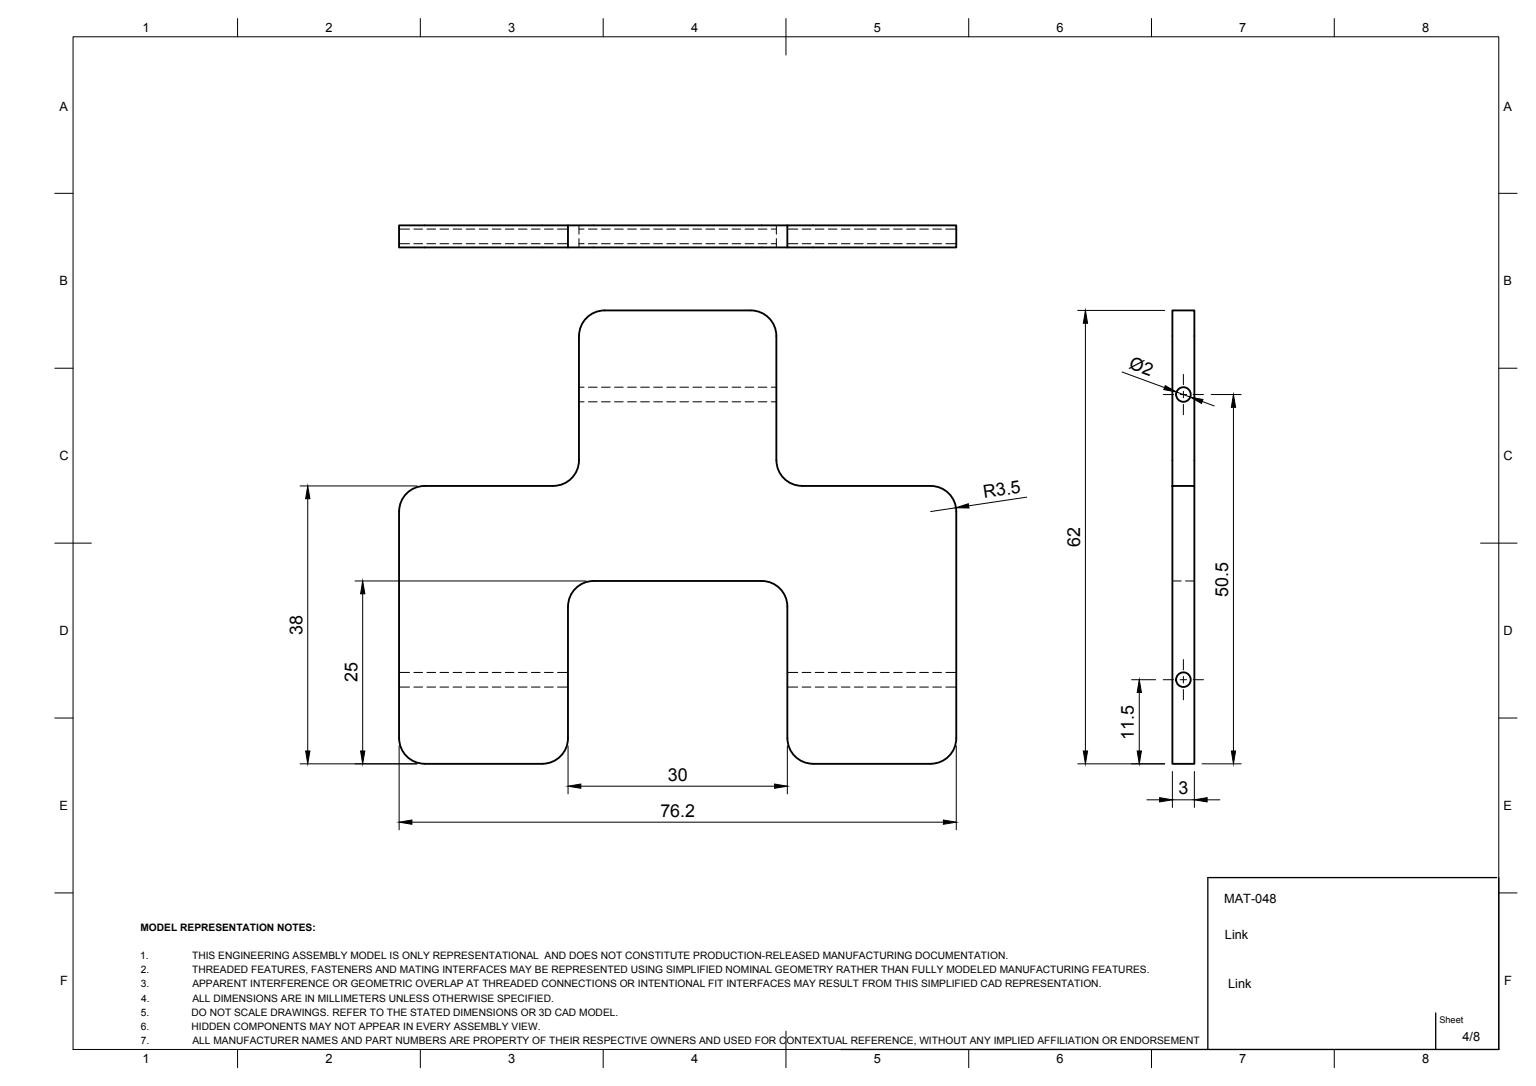
ISO-10303-21;
HEADER;
/* Generated by software containing ST-Developer
 * from STEP Tools, Inc. (www.steptools.com) 
 */

FILE_DESCRIPTION(
/* description */ ('STEP AP214'),
/* implementation_level */ '2;1');

FILE_NAME(
/* name */ 'Link.step',
/* time_stamp */ '2026-11-14T22:24:45-08:00',
/* author */ (''),
/* organization */ (''),
/* preprocessor_version */ 'ST-DEVELOPER v20.2',
/* originating_system */ 'Autodesk Translation Framework v15.17.0.0',
/* authorisation */ '');

FILE_SCHEMA (('AUTOMOTIVE_DESIGN { 1 0 10303 214 3 1 1 }'));
ENDSEC;

DATA;
#10=MECHANICAL_DESIGN_GEOMETRIC_PRESENTATION_REPRESENTATION('',(#129),#5599);
#107=FACE_BOUND('',#614,.T.);
#108=FACE_BOUND('',#619,.T.);
#109=FACE_BOUND('',#624,.T.);
#110=FACE_BOUND('',#629,.T.);
#111=FACE_BOUND('',#634,.T.);
#112=FACE_BOUND('',#639,.T.);
#117=SHAPE_REPRESENTATION_RELATIONSHIP('SRR','None',#5645,#123);
#123=ADVANCED_BREP_SHAPE_REPRESENTATION('',(#135),#5597);
#129=STYLED_ITEM('',(#5680),#135);
#135=MANIFOLD_SOLID_BREP('Body1',#3311);
#177=CYLINDRICAL_SURFACE('',#3594,0.999999999999991);
#178=CYLINDRICAL_SURFACE('',#3597,0.999999999999991);
#179=CYLINDRICAL_SURFACE('',#3600,1.);
#180=CYLINDRICAL_SURFACE('',#3603,3.5);
#181=CYLINDRICAL_SURFACE('',#3607,3.5);
#182=CYLINDRICAL_SURFACE('',#3611,3.5);
#183=CYLINDRICAL_SURFACE('',#3615,3.5);
#184=CYLINDRICAL_SURFACE('',#3619,3.5);
#185=CYLINDRICAL_SURFACE('',#3623,3.5);
#186=CYLINDRICAL_SURFACE('',#3627,3.5);
#187=CYLINDRICAL_SURFACE('',#3631,3.5);
#188=CYLINDRICAL_SURFACE('',#3635,3.5);
#189=CYLINDRICAL_SURFACE('',#3639,3.5);
#190=CYLINDRICAL_SURFACE('',#3643,3.5);
#191=CYLINDRICAL_SURFACE('',#3647,3.5);
#249=CIRCLE('',#3595,0.999999999999991);
#250=CIRCLE('',#3596,0.999999999999991);
#251=CIRCLE('',#3598,0.999999999999991);
#252=CIRCLE('',#3599,0.999999999999991);
#253=CIRCLE('',#3601,0.999999999999988);
#254=CIRCLE('',#3602,1.);
#255=CIRCLE('',#3604,3.5);
#256=CIRCLE('',#3605,3.5);
#257=CIRCLE('',#3608,3.5);
#258=CIRCLE('',#3609,3.5);
#259=CIRCLE('',#3612,3.5);
#260=CIRCLE('',#3613,3.5);
#261=CIRCLE('',#3616,3.5);
#262=CIRCLE('',#3617,3.5);
#263=CIRCLE('',#3620,3.5);
#264=CIRCLE('',#3621,3.5);
#265=CIRCLE('',#3624,3.5);
#266=CIRCLE('',#3625,3.5);
#267=CIRCLE('',#3628,3.5);
#268=CIRCLE('',#3629,3.5);
#269=CIRCLE('',#3632,3.5);
#270=CIRCLE('',#3633,3.5);
#271=CIRCLE('',#3636,3.5);
#272=CIRCLE('',#3637,3.5);
#273=CIRCLE('',#3640,3.5);
#274=CIRCLE('',#3641,3.5);
#275=CIRCLE('',#3644,3.5);
#276=CIRCLE('',#3645,3.5);
#277=CIRCLE('',#3648,3.5);
#278=CIRCLE('',#3649,3.5);
#425=FACE_OUTER_BOUND('',#609,.T.);
#426=FACE_OUTER_BOUND('',#610,.T.);
#427=FACE_OUTER_BOUND('',#611,.T.);
#428=FACE_OUTER_BOUND('',#612,.T.);
#429=FACE_OUTER_BOUND('',#613,.T.);
#430=FACE_OUTER_BOUND('',#615,.T.);
#431=FACE_OUTER_BOUND('',#616,.T.);
#432=FACE_OUTER_BOUND('',#617,.T.);
#433=FACE_OUTER_BOUND('',#618,.T.);
#434=FACE_OUTER_BOUND('',#620,.T.);
#435=FACE_OUTER_BOUND('',#621,.T.);
#436=FACE_OUTER_BOUND('',#622,.T.);
#437=FACE_OUTER_BOUND('',#623,.T.);
#438=FACE_OUTER_BOUND('',#625,.T.);
#439=FACE_OUTER_BOUND('',#626,.T.);
#440=FACE_OUTER_BOUND('',#627,.T.);
#441=FACE_OUTER_BOUND('',#628,.T.);
#442=FACE_OUTER_BOUND('',#630,.T.);
#443=FACE_OUTER_BOUND('',#631,.T.);
#444=FACE_OUTER_BOUND('',#632,.T.);
#445=FACE_OUTER_BOUND('',#633,.T.);
#446=FACE_OUTER_BOUND('',#635,.T.);
#447=FACE_OUTER_BOUND('',#636,.T.);
#448=FACE_OUTER_BOUND('',#637,.T.);
#449=FACE_OUTER_BOUND('',#638,.T.);
#450=FACE_OUTER_BOUND('',#640,.T.);
#451=FACE_OUTER_BOUND('',#641,.T.);
#452=FACE_OUTER_BOUND('',#642,.T.);
#453=FACE_OUTER_BOUND('',#643,.T.);
#609=EDGE_LOOP('',(#2835,#2836,#2837,#2838));
#610=EDGE_LOOP('',(#2839,#2840,#2841,#2842));
#611=EDGE_LOOP('',(#2843,#2844,#2845,#2846));
#612=EDGE_LOOP('',(#2847,#2848,#2849,#2850));
#613=EDGE_LOOP('',(#2851,#2852,#2853,#2854));
#614=EDGE_LOOP('',(#2855));
#615=EDGE_LOOP('',(#2856,#2857,#2858,#2859));
#616=EDGE_LOOP('',(#2860,#2861,#2862,#2863));
#617=EDGE_LOOP('',(#2864,#2865,#2866,#2867));
#618=EDGE_LOOP('',(#2868,#2869,#2870,#2871));
#619=EDGE_LOOP('',(#2872));
#620=EDGE_LOOP('',(#2873,#2874,#2875,#2876));
#621=EDGE_LOOP('',(#2877,#2878,#2879,#2880));
#622=EDGE_LOOP('',(#2881,#2882,#2883,#2884));
#623=EDGE_LOOP('',(#2885,#2886,#2887,#2888));
#624=EDGE_LOOP('',(#2889));
#625=EDGE_LOOP('',(#2890,#2891,#2892,#2893));
#626=EDGE_LOOP('',(#2894,#2895,#2896,#2897));
#627=EDGE_LOOP('',(#2898,#2899,#2900,#2901));
#628=EDGE_LOOP('',(#2902,#2903,#2904,#2905));
#629=EDGE_LOOP('',(#2906));
#630=EDGE_LOOP('',(#2907,#2908,#2909,#2910));
#631=EDGE_LOOP('',(#2911,#2912,#2913,#2914));
#632=EDGE_LOOP('',(#2915,#2916,#2917,#2918));
#633=EDGE_LOOP('',(#2919,#2920,#2921,#2922));
#634=EDGE_LOOP('',(#2923));
#635=EDGE_LOOP('',(#2924,#2925,#2926,#2927));
#636=EDGE_LOOP('',(#2928,#2929,#2930,#2931));
#637=EDGE_LOOP('',(#2932,#2933,#2934,#2935));
#638=EDGE_LOOP('',(#2936,#2937,#2938,#2939));
#639=EDGE_LOOP('',(#2940));
#640=EDGE_LOOP('',(#2941,#2942,#2943,#2944));
#641=EDGE_LOOP('',(#2945,#2946,#2947,#2948));
#642=EDGE_LOOP('',(#2949,#2950,#2951,#2952,#2953,#2954,#2955,#2956,#2957,
#2958,#2959,#2960,#2961,#2962,#2963,#2964,#2965,#2966,#2967,#2968,#2969,
#2970,#2971,#2972));
#643=EDGE_LOOP('',(#2973,#2974,#2975,#2976,#2977,#2978,#2979,#2980,#2981,
#2982,#2983,#2984,#2985,#2986,#2987,#2988,#2989,#2990,#2991,#2992,#2993,
#2994,#2995,#2996));
#951=LINE('',#5393,#1307);
#952=LINE('',#5399,#1308);
#953=LINE('',#5405,#1309);
#954=LINE('',#5412,#1310);
#955=LINE('',#5415,#1311);
#956=LINE('',#5418,#1312);
#957=LINE('',#5420,#1313);
#958=LINE('',#5421,#1314);
#959=LINE('',#5426,#1315);
#960=LINE('',#5430,#1316);
#961=LINE('',#5432,#1317);
#962=LINE('',#5433,#1318);
#963=LINE('',#5438,#1319);
#964=LINE('',#5442,#1320);
#965=LINE('',#5444,#1321);
#966=LINE('',#5445,#1322);
#967=LINE('',#5450,#1323);
#968=LINE('',#5454,#1324);
#969=LINE('',#5456,#1325);
#970=LINE('',#5457,#1326);
#971=LINE('',#5462,#1327);
#972=LINE('',#5466,#1328);
#973=LINE('',#5468,#1329);
#974=LINE('',#5469,#1330);
#975=LINE('',#5474,#1331);
#976=LINE('',#5478,#1332);
#977=LINE('',#5480,#1333);
#978=LINE('',#5481,#1334);
#979=LINE('',#5486,#1335);
#980=LINE('',#5490,#1336);
#981=LINE('',#5492,#1337);
#982=LINE('',#5493,#1338);
#983=LINE('',#5498,#1339);
#984=LINE('',#5502,#1340);
#985=LINE('',#5504,#1341);
#986=LINE('',#5505,#1342);
#987=LINE('',#5510,#1343);
#988=LINE('',#5514,#1344);
#989=LINE('',#5516,#1345);
#990=LINE('',#5517,#1346);
#991=LINE('',#5522,#1347);
#992=LINE('',#5526,#1348);
#993=LINE('',#5528,#1349);
#994=LINE('',#5529,#1350);
#995=LINE('',#5534,#1351);
#996=LINE('',#5538,#1352);
#997=LINE('',#5540,#1353);
#998=LINE('',#5541,#1354);
#999=LINE('',#5546,#1355);
#1000=LINE('',#5549,#1356);
#1001=LINE('',#5550,#1357);
#1307=VECTOR('',#4417,0.999999999999991);
#1308=VECTOR('',#4424,0.999999999999991);
#1309=VECTOR('',#4431,1.);
#1310=VECTOR('',#4438,1000.);
#1311=VECTOR('',#4441,1000.);
#1312=VECTOR('',#4444,1000.);
#1313=VECTOR('',#4445,1000.);
#1314=VECTOR('',#4446,1000.);
#1315=VECTOR('',#4451,1000.);
#1316=VECTOR('',#4456,1000.);
#1317=VECTOR('',#4457,1000.);
#1318=VECTOR('',#4458,1000.);
#1319=VECTOR('',#4463,1000.);
#1320=VECTOR('',#4468,1000.);
#1321=VECTOR('',#4469,1000.);
#1322=VECTOR('',#4470,1000.);
#1323=VECTOR('',#4475,1000.);
#1324=VECTOR('',#4480,1000.);
#1325=VECTOR('',#4481,1000.);
#1326=VECTOR('',#4482,1000.);
#1327=VECTOR('',#4487,1000.);
#1328=VECTOR('',#4492,1000.);
#1329=VECTOR('',#4493,1000.);
#1330=VECTOR('',#4494,1000.);
#1331=VECTOR('',#4499,1000.);
#1332=VECTOR('',#4504,1000.);
#1333=VECTOR('',#4505,1000.);
#1334=VECTOR('',#4506,1000.);
#1335=VECTOR('',#4511,1000.);
#1336=VECTOR('',#4516,1000.);
#1337=VECTOR('',#4517,1000.);
#1338=VECTOR('',#4518,1000.);
#1339=VECTOR('',#4523,1000.);
#1340=VECTOR('',#4528,1000.);
#1341=VECTOR('',#4529,1000.);
#1342=VECTOR('',#4530,1000.);
#1343=VECTOR('',#4535,1000.);
#1344=VECTOR('',#4540,1000.);
#1345=VECTOR('',#4541,1000.);
#1346=VECTOR('',#4542,1000.);
#1347=VECTOR('',#4547,1000.);
#1348=VECTOR('',#4552,1000.);
#1349=VECTOR('',#4553,1000.);
#1350=VECTOR('',#4554,1000.);
#1351=VECTOR('',#4559,1000.);
#1352=VECTOR('',#4564,1000.);
#1353=VECTOR('',#4565,1000.);
#1354=VECTOR('',#4566,1000.);
#1355=VECTOR('',#4571,1000.);
#1356=VECTOR('',#4576,1000.);
#1357=VECTOR('',#4577,1000.);
#1591=VERTEX_POINT('',#5390);
#1592=VERTEX_POINT('',#5392);
#1593=VERTEX_POINT('',#5396);
#1594=VERTEX_POINT('',#5398);
#1595=VERTEX_POINT('',#5402);
#1596=VERTEX_POINT('',#5404);
#1597=VERTEX_POINT('',#5408);
#1598=VERTEX_POINT('',#5409);
#1599=VERTEX_POINT('',#5411);
#1600=VERTEX_POINT('',#5413);
#1601=VERTEX_POINT('',#5417);
#1602=VERTEX_POINT('',#5419);
#1603=VERTEX_POINT('',#5423);
#1604=VERTEX_POINT('',#5425);
#1605=VERTEX_POINT('',#5429);
#1606=VERTEX_POINT('',#5431);
#1607=VERTEX_POINT('',#5435);
#1608=VERTEX_POINT('',#5437);
#1609=VERTEX_POINT('',#5441);
#1610=VERTEX_POINT('',#5443);
#1611=VERTEX_POINT('',#5447);
#1612=VERTEX_POINT('',#5449);
#1613=VERTEX_POINT('',#5453);
#1614=VERTEX_POINT('',#5455);
#1615=VERTEX_POINT('',#5459);
#1616=VERTEX_POINT('',#5461);
#1617=VERTEX_POINT('',#5465);
#1618=VERTEX_POINT('',#5467);
#1619=VERTEX_POINT('',#5471);
#1620=VERTEX_POINT('',#5473);
#1621=VERTEX_POINT('',#5477);
#1622=VERTEX_POINT('',#5479);
#1623=VERTEX_POINT('',#5483);
#1624=VERTEX_POINT('',#5485);
#1625=VERTEX_POINT('',#5489);
#1626=VERTEX_POINT('',#5491);
#1627=VERTEX_POINT('',#5495);
#1628=VERTEX_POINT('',#5497);
#1629=VERTEX_POINT('',#5501);
#1630=VERTEX_POINT('',#5503);
#1631=VERTEX_POINT('',#5507);
#1632=VERTEX_POINT('',#5509);
#1633=VERTEX_POINT('',#5513);
#1634=VERTEX_POINT('',#5515);
#1635=VERTEX_POINT('',#5519);
#1636=VERTEX_POINT('',#5521);
#1637=VERTEX_POINT('',#5525);
#1638=VERTEX_POINT('',#5527);
#1639=VERTEX_POINT('',#5531);
#1640=VERTEX_POINT('',#5533);
#1641=VERTEX_POINT('',#5537);
#1642=VERTEX_POINT('',#5539);
#1643=VERTEX_POINT('',#5543);
#1644=VERTEX_POINT('',#5545);
#2015=EDGE_CURVE('',#1591,#1591,#249,.T.);
#2016=EDGE_CURVE('',#1591,#1592,#951,.T.);
#2017=EDGE_CURVE('',#1592,#1592,#250,.T.);
#2018=EDGE_CURVE('',#1593,#1593,#251,.T.);
#2019=EDGE_CURVE('',#1593,#1594,#952,.T.);
#2020=EDGE_CURVE('',#1594,#1594,#252,.T.);
#2021=EDGE_CURVE('',#1595,#1595,#253,.T.);
#2022=EDGE_CURVE('',#1595,#1596,#953,.T.);
#2023=EDGE_CURVE('',#1596,#1596,#254,.T.);
#2024=EDGE_CURVE('',#1597,#1598,#255,.T.);
#2025=EDGE_CURVE('',#1599,#1598,#954,.T.);
#2026=EDGE_CURVE('',#1600,#1599,#256,.T.);
#2027=EDGE_CURVE('',#1600,#1597,#955,.T.);
#2028=EDGE_CURVE('',#1598,#1601,#956,.T.);
#2029=EDGE_CURVE('',#1602,#1601,#957,.T.);
#2030=EDGE_CURVE('',#1599,#1602,#958,.T.);
#2031=EDGE_CURVE('',#1601,#1603,#257,.T.);
#2032=EDGE_CURVE('',#1604,#1603,#959,.T.);
#2033=EDGE_CURVE('',#1602,#1604,#258,.T.);
#2034=EDGE_CURVE('',#1603,#1605,#960,.T.);
#2035=EDGE_CURVE('',#1606,#1605,#961,.T.);
#2036=EDGE_CURVE('',#1604,#1606,#962,.T.);
#2037=EDGE_CURVE('',#1605,#1607,#259,.T.);
#2038=EDGE_CURVE('',#1608,#1607,#963,.T.);
#2039=EDGE_CURVE('',#1606,#1608,#260,.T.);
#2040=EDGE_CURVE('',#1607,#1609,#964,.T.);
#2041=EDGE_CURVE('',#1610,#1609,#965,.T.);
#2042=EDGE_CURVE('',#1608,#1610,#966,.T.);
#2043=EDGE_CURVE('',#1609,#1611,#261,.T.);
#2044=EDGE_CURVE('',#1612,#1611,#967,.T.);
#2045=EDGE_CURVE('',#1610,#1612,#262,.T.);
#2046=EDGE_CURVE('',#1611,#1613,#968,.T.);
#2047=EDGE_CURVE('',#1614,#1613,#969,.T.);
#2048=EDGE_CURVE('',#1612,#1614,#970,.T.);
#2049=EDGE_CURVE('',#1613,#1615,#263,.T.);
#2050=EDGE_CURVE('',#1616,#1615,#971,.T.);
#2051=EDGE_CURVE('',#1614,#1616,#264,.T.);
#2052=EDGE_CURVE('',#1615,#1617,#972,.T.);
#2053=EDGE_CURVE('',#1618,#1617,#973,.T.);
#2054=EDGE_CURVE('',#1616,#1618,#974,.T.);
#2055=EDGE_CURVE('',#1617,#1619,#265,.T.);
#2056=EDGE_CURVE('',#1620,#1619,#975,.T.);
#2057=EDGE_CURVE('',#1618,#1620,#266,.T.);
#2058=EDGE_CURVE('',#1619,#1621,#976,.T.);
#2059=EDGE_CURVE('',#1622,#1621,#977,.T.);
#2060=EDGE_CURVE('',#1620,#1622,#978,.T.);
#2061=EDGE_CURVE('',#1621,#1623,#267,.T.);
#2062=EDGE_CURVE('',#1624,#1623,#979,.T.);
#2063=EDGE_CURVE('',#1622,#1624,#268,.T.);
#2064=EDGE_CURVE('',#1623,#1625,#980,.T.);
#2065=EDGE_CURVE('',#1626,#1625,#981,.T.);
#2066=EDGE_CURVE('',#1624,#1626,#982,.T.);
#2067=EDGE_CURVE('',#1625,#1627,#269,.T.);
#2068=EDGE_CURVE('',#1628,#1627,#983,.T.);
#2069=EDGE_CURVE('',#1626,#1628,#270,.T.);
#2070=EDGE_CURVE('',#1627,#1629,#984,.T.);
#2071=EDGE_CURVE('',#1630,#1629,#985,.T.);
#2072=EDGE_CURVE('',#1628,#1630,#986,.T.);
#2073=EDGE_CURVE('',#1629,#1631,#271,.T.);
#2074=EDGE_CURVE('',#1632,#1631,#987,.T.);
#2075=EDGE_CURVE('',#1630,#1632,#272,.T.);
#2076=EDGE_CURVE('',#1631,#1633,#988,.T.);
#2077=EDGE_CURVE('',#1634,#1633,#989,.T.);
#2078=EDGE_CURVE('',#1632,#1634,#990,.T.);
#2079=EDGE_CURVE('',#1633,#1635,#273,.T.);
#2080=EDGE_CURVE('',#1636,#1635,#991,.T.);
#2081=EDGE_CURVE('',#1634,#1636,#274,.T.);
#2082=EDGE_CURVE('',#1635,#1637,#992,.T.);
#2083=EDGE_CURVE('',#1638,#1637,#993,.T.);
#2084=EDGE_CURVE('',#1636,#1638,#994,.T.);
#2085=EDGE_CURVE('',#1637,#1639,#275,.T.);
#2086=EDGE_CURVE('',#1640,#1639,#995,.T.);
#2087=EDGE_CURVE('',#1638,#1640,#276,.T.);
#2088=EDGE_CURVE('',#1639,#1641,#996,.T.);
#2089=EDGE_CURVE('',#1642,#1641,#997,.T.);
#2090=EDGE_CURVE('',#1640,#1642,#998,.T.);
#2091=EDGE_CURVE('',#1641,#1643,#277,.T.);
#2092=EDGE_CURVE('',#1644,#1643,#999,.T.);
#2093=EDGE_CURVE('',#1642,#1644,#278,.T.);
#2094=EDGE_CURVE('',#1643,#1597,#1000,.T.);
#2095=EDGE_CURVE('',#1644,#1600,#1001,.T.);
#2835=ORIENTED_EDGE('',*,*,#2015,.F.);
#2836=ORIENTED_EDGE('',*,*,#2016,.T.);
#2837=ORIENTED_EDGE('',*,*,#2017,.F.);
#2838=ORIENTED_EDGE('',*,*,#2016,.F.);
#2839=ORIENTED_EDGE('',*,*,#2018,.F.);
#2840=ORIENTED_EDGE('',*,*,#2019,.T.);
#2841=ORIENTED_EDGE('',*,*,#2020,.T.);
#2842=ORIENTED_EDGE('',*,*,#2019,.F.);
#2843=ORIENTED_EDGE('',*,*,#2021,.F.);
#2844=ORIENTED_EDGE('',*,*,#2022,.T.);
#2845=ORIENTED_EDGE('',*,*,#2023,.T.);
#2846=ORIENTED_EDGE('',*,*,#2022,.F.);
#2847=ORIENTED_EDGE('',*,*,#2024,.T.);
#2848=ORIENTED_EDGE('',*,*,#2025,.F.);
#2849=ORIENTED_EDGE('',*,*,#2026,.F.);
#2850=ORIENTED_EDGE('',*,*,#2027,.T.);
#2851=ORIENTED_EDGE('',*,*,#2028,.T.);
#2852=ORIENTED_EDGE('',*,*,#2029,.F.);
#2853=ORIENTED_EDGE('',*,*,#2030,.F.);
#2854=ORIENTED_EDGE('',*,*,#2025,.T.);
#2855=ORIENTED_EDGE('',*,*,#2018,.T.);
#2856=ORIENTED_EDGE('',*,*,#2031,.T.);
#2857=ORIENTED_EDGE('',*,*,#2032,.F.);
#2858=ORIENTED_EDGE('',*,*,#2033,.F.);
#2859=ORIENTED_EDGE('',*,*,#2029,.T.);
#2860=ORIENTED_EDGE('',*,*,#2034,.T.);
#2861=ORIENTED_EDGE('',*,*,#2035,.F.);
#2862=ORIENTED_EDGE('',*,*,#2036,.F.);
#2863=ORIENTED_EDGE('',*,*,#2032,.T.);
#2864=ORIENTED_EDGE('',*,*,#2037,.T.);
#2865=ORIENTED_EDGE('',*,*,#2038,.F.);
#2866=ORIENTED_EDGE('',*,*,#2039,.F.);
#2867=ORIENTED_EDGE('',*,*,#2035,.T.);
#2868=ORIENTED_EDGE('',*,*,#2040,.T.);
#2869=ORIENTED_EDGE('',*,*,#2041,.F.);
#2870=ORIENTED_EDGE('',*,*,#2042,.F.);
#2871=ORIENTED_EDGE('',*,*,#2038,.T.);
#2872=ORIENTED_EDGE('',*,*,#2017,.T.);
#2873=ORIENTED_EDGE('',*,*,#2043,.T.);
#2874=ORIENTED_EDGE('',*,*,#2044,.F.);
#2875=ORIENTED_EDGE('',*,*,#2045,.F.);
#2876=ORIENTED_EDGE('',*,*,#2041,.T.);
#2877=ORIENTED_EDGE('',*,*,#2046,.T.);
#2878=ORIENTED_EDGE('',*,*,#2047,.F.);
#2879=ORIENTED_EDGE('',*,*,#2048,.F.);
#2880=ORIENTED_EDGE('',*,*,#2044,.T.);
#2881=ORIENTED_EDGE('',*,*,#2049,.T.);
#2882=ORIENTED_EDGE('',*,*,#2050,.F.);
#2883=ORIENTED_EDGE('',*,*,#2051,.F.);
#2884=ORIENTED_EDGE('',*,*,#2047,.T.);
#2885=ORIENTED_EDGE('',*,*,#2052,.T.);
#2886=ORIENTED_EDGE('',*,*,#2053,.F.);
#2887=ORIENTED_EDGE('',*,*,#2054,.F.);
#2888=ORIENTED_EDGE('',*,*,#2050,.T.);
#2889=ORIENTED_EDGE('',*,*,#2015,.T.);
#2890=ORIENTED_EDGE('',*,*,#2055,.T.);
#2891=ORIENTED_EDGE('',*,*,#2056,.F.);
#2892=ORIENTED_EDGE('',*,*,#2057,.F.);
#2893=ORIENTED_EDGE('',*,*,#2053,.T.);
#2894=ORIENTED_EDGE('',*,*,#2058,.T.);
#2895=ORIENTED_EDGE('',*,*,#2059,.F.);
#2896=ORIENTED_EDGE('',*,*,#2060,.F.);
#2897=ORIENTED_EDGE('',*,*,#2056,.T.);
#2898=ORIENTED_EDGE('',*,*,#2061,.T.);
#2899=ORIENTED_EDGE('',*,*,#2062,.F.);
#2900=ORIENTED_EDGE('',*,*,#2063,.F.);
#2901=ORIENTED_EDGE('',*,*,#2059,.T.);
#2902=ORIENTED_EDGE('',*,*,#2064,.T.);
#2903=ORIENTED_EDGE('',*,*,#2065,.F.);
#2904=ORIENTED_EDGE('',*,*,#2066,.F.);
#2905=ORIENTED_EDGE('',*,*,#2062,.T.);
#2906=ORIENTED_EDGE('',*,*,#2021,.T.);
#2907=ORIENTED_EDGE('',*,*,#2067,.T.);
#2908=ORIENTED_EDGE('',*,*,#2068,.F.);
#2909=ORIENTED_EDGE('',*,*,#2069,.F.);
#2910=ORIENTED_EDGE('',*,*,#2065,.T.);
#2911=ORIENTED_EDGE('',*,*,#2070,.T.);
#2912=ORIENTED_EDGE('',*,*,#2071,.F.);
#2913=ORIENTED_EDGE('',*,*,#2072,.F.);
#2914=ORIENTED_EDGE('',*,*,#2068,.T.);
#2915=ORIENTED_EDGE('',*,*,#2073,.T.);
#2916=ORIENTED_EDGE('',*,*,#2074,.F.);
#2917=ORIENTED_EDGE('',*,*,#2075,.F.);
#2918=ORIENTED_EDGE('',*,*,#2071,.T.);
#2919=ORIENTED_EDGE('',*,*,#2076,.T.);
#2920=ORIENTED_EDGE('',*,*,#2077,.F.);
#2921=ORIENTED_EDGE('',*,*,#2078,.F.);
#2922=ORIENTED_EDGE('',*,*,#2074,.T.);
#2923=ORIENTED_EDGE('',*,*,#2023,.F.);
#2924=ORIENTED_EDGE('',*,*,#2079,.T.);
#2925=ORIENTED_EDGE('',*,*,#2080,.F.);
#2926=ORIENTED_EDGE('',*,*,#2081,.F.);
#2927=ORIENTED_EDGE('',*,*,#2077,.T.);
#2928=ORIENTED_EDGE('',*,*,#2082,.T.);
#2929=ORIENTED_EDGE('',*,*,#2083,.F.);
#2930=ORIENTED_EDGE('',*,*,#2084,.F.);
#2931=ORIENTED_EDGE('',*,*,#2080,.T.);
#2932=ORIENTED_EDGE('',*,*,#2085,.T.);
#2933=ORIENTED_EDGE('',*,*,#2086,.F.);
#2934=ORIENTED_EDGE('',*,*,#2087,.F.);
#2935=ORIENTED_EDGE('',*,*,#2083,.T.);
#2936=ORIENTED_EDGE('',*,*,#2088,.T.);
#2937=ORIENTED_EDGE('',*,*,#2089,.F.);
#2938=ORIENTED_EDGE('',*,*,#2090,.F.);
#2939=ORIENTED_EDGE('',*,*,#2086,.T.);
#2940=ORIENTED_EDGE('',*,*,#2020,.F.);
#2941=ORIENTED_EDGE('',*,*,#2091,.T.);
#2942=ORIENTED_EDGE('',*,*,#2092,.F.);
#2943=ORIENTED_EDGE('',*,*,#2093,.F.);
#2944=ORIENTED_EDGE('',*,*,#2089,.T.);
#2945=ORIENTED_EDGE('',*,*,#2094,.T.);
#2946=ORIENTED_EDGE('',*,*,#2027,.F.);
#2947=ORIENTED_EDGE('',*,*,#2095,.F.);
#2948=ORIENTED_EDGE('',*,*,#2092,.T.);
#2949=ORIENTED_EDGE('',*,*,#2026,.T.);
#2950=ORIENTED_EDGE('',*,*,#2030,.T.);
#2951=ORIENTED_EDGE('',*,*,#2033,.T.);
#2952=ORIENTED_EDGE('',*,*,#2036,.T.);
#2953=ORIENTED_EDGE('',*,*,#2039,.T.);
#2954=ORIENTED_EDGE('',*,*,#2042,.T.);
#2955=ORIENTED_EDGE('',*,*,#2045,.T.);
#2956=ORIENTED_EDGE('',*,*,#2048,.T.);
#2957=ORIENTED_EDGE('',*,*,#2051,.T.);
#2958=ORIENTED_EDGE('',*,*,#2054,.T.);
#2959=ORIENTED_EDGE('',*,*,#2057,.T.);
#2960=ORIENTED_EDGE('',*,*,#2060,.T.);
#2961=ORIENTED_EDGE('',*,*,#2063,.T.);
#2962=ORIENTED_EDGE('',*,*,#2066,.T.);
#2963=ORIENTED_EDGE('',*,*,#2069,.T.);
#2964=ORIENTED_EDGE('',*,*,#2072,.T.);
#2965=ORIENTED_EDGE('',*,*,#2075,.T.);
#2966=ORIENTED_EDGE('',*,*,#2078,.T.);
#2967=ORIENTED_EDGE('',*,*,#2081,.T.);
#2968=ORIENTED_EDGE('',*,*,#2084,.T.);
#2969=ORIENTED_EDGE('',*,*,#2087,.T.);
#2970=ORIENTED_EDGE('',*,*,#2090,.T.);
#2971=ORIENTED_EDGE('',*,*,#2093,.T.);
#2972=ORIENTED_EDGE('',*,*,#2095,.T.);
#2973=ORIENTED_EDGE('',*,*,#2024,.F.);
#2974=ORIENTED_EDGE('',*,*,#2094,.F.);
#2975=ORIENTED_EDGE('',*,*,#2091,.F.);
#2976=ORIENTED_EDGE('',*,*,#2088,.F.);
#2977=ORIENTED_EDGE('',*,*,#2085,.F.);
#2978=ORIENTED_EDGE('',*,*,#2082,.F.);
#2979=ORIENTED_EDGE('',*,*,#2079,.F.);
#2980=ORIENTED_EDGE('',*,*,#2076,.F.);
#2981=ORIENTED_EDGE('',*,*,#2073,.F.);
#2982=ORIENTED_EDGE('',*,*,#2070,.F.);
#2983=ORIENTED_EDGE('',*,*,#2067,.F.);
#2984=ORIENTED_EDGE('',*,*,#2064,.F.);
#2985=ORIENTED_EDGE('',*,*,#2061,.F.);
#2986=ORIENTED_EDGE('',*,*,#2058,.F.);
#2987=ORIENTED_EDGE('',*,*,#2055,.F.);
#2988=ORIENTED_EDGE('',*,*,#2052,.F.);
#2989=ORIENTED_EDGE('',*,*,#2049,.F.);
#2990=ORIENTED_EDGE('',*,*,#2046,.F.);
#2991=ORIENTED_EDGE('',*,*,#2043,.F.);
#2992=ORIENTED_EDGE('',*,*,#2040,.F.);
#2993=ORIENTED_EDGE('',*,*,#2037,.F.);
#2994=ORIENTED_EDGE('',*,*,#2034,.F.);
#2995=ORIENTED_EDGE('',*,*,#2031,.F.);
#2996=ORIENTED_EDGE('',*,*,#2028,.F.);
#3115=PLANE('',#3606);
#3116=PLANE('',#3610);
#3117=PLANE('',#3614);
#3118=PLANE('',#3618);
#3119=PLANE('',#3622);
#3120=PLANE('',#3626);
#3121=PLANE('',#3630);
#3122=PLANE('',#3634);
#3123=PLANE('',#3638);
#3124=PLANE('',#3642);
#3125=PLANE('',#3646);
#3126=PLANE('',#3650);
#3127=PLANE('',#3651);
#3128=PLANE('',#3652);
#3275=ADVANCED_FACE('',(#425),#177,.F.);
#3276=ADVANCED_FACE('',(#426),#178,.F.);
#3277=ADVANCED_FACE('',(#427),#179,.F.);
#3278=ADVANCED_FACE('',(#428),#180,.T.);
#3279=ADVANCED_FACE('',(#429,#107),#3115,.F.);
#3280=ADVANCED_FACE('',(#430),#181,.F.);
#3281=ADVANCED_FACE('',(#431),#3116,.F.);
#3282=ADVANCED_FACE('',(#432),#182,.F.);
#3283=ADVANCED_FACE('',(#433,#108),#3117,.F.);
#3284=ADVANCED_FACE('',(#434),#183,.T.);
#3285=ADVANCED_FACE('',(#435),#3118,.F.);
#3286=ADVANCED_FACE('',(#436),#184,.T.);
#3287=ADVANCED_FACE('',(#437,#109),#3119,.F.);
#3288=ADVANCED_FACE('',(#438),#185,.T.);
#3289=ADVANCED_FACE('',(#439),#3120,.F.);
#3290=ADVANCED_FACE('',(#440),#186,.F.);
#3291=ADVANCED_FACE('',(#441,#110),#3121,.F.);
#3292=ADVANCED_FACE('',(#442),#187,.T.);
#3293=ADVANCED_FACE('',(#443),#3122,.F.);
#3294=ADVANCED_FACE('',(#444),#188,.T.);
#3295=ADVANCED_FACE('',(#445,#111),#3123,.F.);
#3296=ADVANCED_FACE('',(#446),#189,.F.);
#3297=ADVANCED_FACE('',(#447),#3124,.F.);
#3298=ADVANCED_FACE('',(#448),#190,.T.);
#3299=ADVANCED_FACE('',(#449,#112),#3125,.F.);
#3300=ADVANCED_FACE('',(#450),#191,.T.);
#3301=ADVANCED_FACE('',(#451),#3126,.F.);
#3302=ADVANCED_FACE('',(#452),#3127,.F.);
#3303=ADVANCED_FACE('',(#453),#3128,.T.);
#3311=CLOSED_SHELL('',(#3275,#3276,#3277,#3278,#3279,#3280,#3281,#3282,
#3283,#3284,#3285,#3286,#3287,#3288,#3289,#3290,#3291,#3292,#3293,#3294,
#3295,#3296,#3297,#3298,#3299,#3300,#3301,#3302,#3303));
#3593=AXIS2_PLACEMENT_3D('',#5388,#4411,#4412);
#3594=AXIS2_PLACEMENT_3D('',#5389,#4413,#4414);
#3595=AXIS2_PLACEMENT_3D('',#5391,#4415,#4416);
#3596=AXIS2_PLACEMENT_3D('',#5394,#4418,#4419);
#3597=AXIS2_PLACEMENT_3D('',#5395,#4420,#4421);
#3598=AXIS2_PLACEMENT_3D('',#5397,#4422,#4423);
#3599=AXIS2_PLACEMENT_3D('',#5400,#4425,#4426);
#3600=AXIS2_PLACEMENT_3D('',#5401,#4427,#4428);
#3601=AXIS2_PLACEMENT_3D('',#5403,#4429,#4430);
#3602=AXIS2_PLACEMENT_3D('',#5406,#4432,#4433);
#3603=AXIS2_PLACEMENT_3D('',#5407,#4434,#4435);
#3604=AXIS2_PLACEMENT_3D('',#5410,#4436,#4437);
#3605=AXIS2_PLACEMENT_3D('',#5414,#4439,#4440);
#3606=AXIS2_PLACEMENT_3D('',#5416,#4442,#4443);
#3607=AXIS2_PLACEMENT_3D('',#5422,#4447,#4448);
#3608=AXIS2_PLACEMENT_3D('',#5424,#4449,#4450);
#3609=AXIS2_PLACEMENT_3D('',#5427,#4452,#4453);
#3610=AXIS2_PLACEMENT_3D('',#5428,#4454,#4455);
#3611=AXIS2_PLACEMENT_3D('',#5434,#4459,#4460);
#3612=AXIS2_PLACEMENT_3D('',#5436,#4461,#4462);
#3613=AXIS2_PLACEMENT_3D('',#5439,#4464,#4465);
#3614=AXIS2_PLACEMENT_3D('',#5440,#4466,#4467);
#3615=AXIS2_PLACEMENT_3D('',#5446,#4471,#4472);
#3616=AXIS2_PLACEMENT_3D('',#5448,#4473,#4474);
#3617=AXIS2_PLACEMENT_3D('',#5451,#4476,#4477);
#3618=AXIS2_PLACEMENT_3D('',#5452,#4478,#4479);
#3619=AXIS2_PLACEMENT_3D('',#5458,#4483,#4484);
#3620=AXIS2_PLACEMENT_3D('',#5460,#4485,#4486);
#3621=AXIS2_PLACEMENT_3D('',#5463,#4488,#4489);
#3622=AXIS2_PLACEMENT_3D('',#5464,#4490,#4491);
#3623=AXIS2_PLACEMENT_3D('',#5470,#4495,#4496);
#3624=AXIS2_PLACEMENT_3D('',#5472,#4497,#4498);
#3625=AXIS2_PLACEMENT_3D('',#5475,#4500,#4501);
#3626=AXIS2_PLACEMENT_3D('',#5476,#4502,#4503);
#3627=AXIS2_PLACEMENT_3D('',#5482,#4507,#4508);
#3628=AXIS2_PLACEMENT_3D('',#5484,#4509,#4510);
#3629=AXIS2_PLACEMENT_3D('',#5487,#4512,#4513);
#3630=AXIS2_PLACEMENT_3D('',#5488,#4514,#4515);
#3631=AXIS2_PLACEMENT_3D('',#5494,#4519,#4520);
#3632=AXIS2_PLACEMENT_3D('',#5496,#4521,#4522);
#3633=AXIS2_PLACEMENT_3D('',#5499,#4524,#4525);
#3634=AXIS2_PLACEMENT_3D('',#5500,#4526,#4527);
#3635=AXIS2_PLACEMENT_3D('',#5506,#4531,#4532);
#3636=AXIS2_PLACEMENT_3D('',#5508,#4533,#4534);
#3637=AXIS2_PLACEMENT_3D('',#5511,#4536,#4537);
#3638=AXIS2_PLACEMENT_3D('',#5512,#4538,#4539);
#3639=AXIS2_PLACEMENT_3D('',#5518,#4543,#4544);
#3640=AXIS2_PLACEMENT_3D('',#5520,#4545,#4546);
#3641=AXIS2_PLACEMENT_3D('',#5523,#4548,#4549);
#3642=AXIS2_PLACEMENT_3D('',#5524,#4550,#4551);
#3643=AXIS2_PLACEMENT_3D('',#5530,#4555,#4556);
#3644=AXIS2_PLACEMENT_3D('',#5532,#4557,#4558);
#3645=AXIS2_PLACEMENT_3D('',#5535,#4560,#4561);
#3646=AXIS2_PLACEMENT_3D('',#5536,#4562,#4563);
#3647=AXIS2_PLACEMENT_3D('',#5542,#4567,#4568);
#3648=AXIS2_PLACEMENT_3D('',#5544,#4569,#4570);
#3649=AXIS2_PLACEMENT_3D('',#5547,#4572,#4573);
#3650=AXIS2_PLACEMENT_3D('',#5548,#4574,#4575);
#3651=AXIS2_PLACEMENT_3D('',#5551,#4578,#4579);
#3652=AXIS2_PLACEMENT_3D('',#5552,#4580,#4581);
#4411=DIRECTION('axis',(0.,0.,1.));
#4412=DIRECTION('refdir',(1.,0.,0.));
#4413=DIRECTION('center_axis',(1.04083408558608E-15,1.,-2.48267427335006E-18));
#4414=DIRECTION('ref_axis',(5.16810401422229E-33,2.48267427335006E-18,1.));
#4415=DIRECTION('center_axis',(1.04083408558608E-15,1.,-2.48267427335006E-18));
#4416=DIRECTION('ref_axis',(5.16810401422229E-33,2.48267427335006E-18,1.));
#4417=DIRECTION('',(1.04083408558608E-15,1.,-2.48267427335006E-18));
#4418=DIRECTION('center_axis',(-1.04083408558608E-15,-1.,2.48267427335006E-18));
#4419=DIRECTION('ref_axis',(-2.58405200711041E-33,-2.48267427335006E-18,
-1.));
#4420=DIRECTION('center_axis',(1.04083408558608E-15,1.,-2.48267427335006E-18));
#4421=DIRECTION('ref_axis',(5.16810401422229E-33,2.48267427335006E-18,1.));
#4422=DIRECTION('center_axis',(1.04083408558608E-15,1.,-2.48267427335006E-18));
#4423=DIRECTION('ref_axis',(2.58405200711041E-33,2.48267427335006E-18,1.));
#4424=DIRECTION('',(1.04083408558608E-15,1.,-2.48267427335006E-18));
#4425=DIRECTION('center_axis',(1.04083408558608E-15,1.,-2.48267427335006E-18));
#4426=DIRECTION('ref_axis',(2.58405200711041E-33,2.48267427335006E-18,1.));
#4427=DIRECTION('center_axis',(1.44900431522769E-15,1.,-2.48267427335006E-18));
#4428=DIRECTION('ref_axis',(-1.,1.44900431522769E-15,-5.16810401422082E-33));
#4429=DIRECTION('center_axis',(1.04083408558608E-15,1.,-2.48267427335006E-18));
#4430=DIRECTION('ref_axis',(2.58405200711041E-33,2.48267427335006E-18,1.));
#4431=DIRECTION('',(1.44900431522769E-15,1.,-2.48267427335006E-18));
#4432=DIRECTION('center_axis',(1.44900431522769E-15,1.,-2.48267427335006E-18));
#4433=DIRECTION('ref_axis',(-1.,1.44900431522769E-15,-3.597405735389E-33));
#4434=DIRECTION('center_axis',(-5.64652480907605E-21,2.48267427335009E-18,
-1.));
#4435=DIRECTION('ref_axis',(-1.,-1.98254111540207E-15,5.64652480907112E-21));
#4436=DIRECTION('center_axis',(5.64652480907605E-21,-2.48267427335009E-18,
1.));
#4437=DIRECTION('ref_axis',(-1.,-1.98254111540207E-15,5.64652480907112E-21));
#4438=DIRECTION('',(-5.64652480907605E-21,2.48267427335009E-18,-1.));
#4439=DIRECTION('center_axis',(5.64652480907605E-21,-2.48267427335009E-18,
1.));
#4440=DIRECTION('ref_axis',(-1.,-1.98254111540207E-15,5.64652480907112E-21));
#4441=DIRECTION('',(-5.64652480907605E-21,2.48267427335009E-18,-1.));
#4442=DIRECTION('center_axis',(1.04083408558608E-15,1.,2.48267427335009E-18));
#4443=DIRECTION('ref_axis',(5.64652480907605E-21,-2.48267427335009E-18,
1.));
#4444=DIRECTION('',(1.,1.04083408558608E-15,5.64652480907598E-21));
#4445=DIRECTION('',(-5.64652480907605E-21,2.48267427335009E-18,-1.));
#4446=DIRECTION('',(1.,1.04083408558608E-15,5.64652480907598E-21));
#4447=DIRECTION('center_axis',(-5.64652480907605E-21,2.48267427335009E-18,
-1.));
#4448=DIRECTION('ref_axis',(-1.,-1.98254111540207E-15,5.64652480907112E-21));
#4449=DIRECTION('center_axis',(-5.64652480907605E-21,2.48267427335009E-18,
-1.));
#4450=DIRECTION('ref_axis',(1.,1.98254111540207E-15,-5.64652480907112E-21));
#4451=DIRECTION('',(-5.64652480907605E-21,2.48267427335009E-18,-1.));
#4452=DIRECTION('center_axis',(-5.64652480907605E-21,2.48267427335009E-18,
-1.));
#4453=DIRECTION('ref_axis',(1.,1.98254111540207E-15,-5.64652480907112E-21));
#4454=DIRECTION('center_axis',(1.,1.04083408558608E-15,-5.64652480907346E-21));
#4455=DIRECTION('ref_axis',(-5.64652480907605E-21,2.48267427335009E-18,
-1.));
#4456=DIRECTION('',(-1.04083408558608E-15,-1.,2.48267427335006E-18));
#4457=DIRECTION('',(-5.64652480907605E-21,2.48267427335009E-18,-1.));
#4458=DIRECTION('',(-1.04083408558608E-15,-1.,2.48267427335006E-18));
#4459=DIRECTION('center_axis',(-5.64652480907605E-21,2.48267427335009E-18,
-1.));
#4460=DIRECTION('ref_axis',(-1.,-9.91270557701033E-16,5.64652480907359E-21));
#4461=DIRECTION('center_axis',(-5.64652480907605E-21,2.48267427335009E-18,
-1.));
#4462=DIRECTION('ref_axis',(1.,9.91270557701033E-16,-5.64652480907359E-21));
#4463=DIRECTION('',(-5.64652480907605E-21,2.48267427335009E-18,-1.));
#4464=DIRECTION('center_axis',(-5.64652480907605E-21,2.48267427335009E-18,
-1.));
#4465=DIRECTION('ref_axis',(1.,9.91270557701033E-16,-5.64652480907359E-21));
#4466=DIRECTION('center_axis',(-1.04083408558608E-15,-1.,-2.48267427335009E-18));
#4467=DIRECTION('ref_axis',(-5.64652480907605E-21,2.48267427335009E-18,
-1.));
#4468=DIRECTION('',(-1.,-1.04083408558608E-15,-5.64652480907598E-21));
#4469=DIRECTION('',(-5.64652480907605E-21,2.48267427335009E-18,-1.));
#4470=DIRECTION('',(-1.,-1.04083408558608E-15,-5.64652480907598E-21));
#4471=DIRECTION('center_axis',(-5.64652480907605E-21,2.48267427335009E-18,
-1.));
#4472=DIRECTION('ref_axis',(-1.,-9.91270557701033E-16,5.64652480907359E-21));
#4473=DIRECTION('center_axis',(5.64652480907605E-21,-2.48267427335009E-18,
1.));
#4474=DIRECTION('ref_axis',(-1.,-9.91270557701033E-16,5.64652480907359E-21));
#4475=DIRECTION('',(-5.64652480907605E-21,2.48267427335009E-18,-1.));
#4476=DIRECTION('center_axis',(5.64652480907605E-21,-2.48267427335009E-18,
1.));
#4477=DIRECTION('ref_axis',(-1.,-9.91270557701033E-16,5.64652480907359E-21));
#4478=DIRECTION('center_axis',(1.,1.04083408558608E-15,-5.64652480907346E-21));
#4479=DIRECTION('ref_axis',(-5.64652480907605E-21,2.48267427335009E-18,
-1.));
#4480=DIRECTION('',(-1.04083408558608E-15,-1.,2.48267427335006E-18));
#4481=DIRECTION('',(-5.64652480907605E-21,2.48267427335009E-18,-1.));
#4482=DIRECTION('',(-1.04083408558608E-15,-1.,2.48267427335006E-18));
#4483=DIRECTION('center_axis',(-5.64652480907605E-21,2.48267427335009E-18,
-1.));
#4484=DIRECTION('ref_axis',(-1.,-9.91270557701033E-16,5.64652480907359E-21));
#4485=DIRECTION('center_axis',(5.64652480907605E-21,-2.48267427335009E-18,
1.));
#4486=DIRECTION('ref_axis',(1.,9.91270557701033E-16,-5.64652480907359E-21));
#4487=DIRECTION('',(-5.64652480907605E-21,2.48267427335009E-18,-1.));
#4488=DIRECTION('center_axis',(5.64652480907605E-21,-2.48267427335009E-18,
1.));
#4489=DIRECTION('ref_axis',(1.,9.91270557701033E-16,-5.64652480907359E-21));
#4490=DIRECTION('center_axis',(-9.84875263780381E-16,1.,-2.48267427335006E-18));
#4491=DIRECTION('ref_axis',(-1.,-9.84875263780381E-16,-5.64652480907612E-21));
#4492=DIRECTION('',(1.,9.84875263780381E-16,5.64652480907612E-21));
#4493=DIRECTION('',(-5.64652480907605E-21,2.48267427335009E-18,-1.));
#4494=DIRECTION('',(1.,9.84875263780381E-16,5.64652480907612E-21));
#4495=DIRECTION('center_axis',(-5.64652480907605E-21,2.48267427335009E-18,
-1.));
#4496=DIRECTION('ref_axis',(-1.,-9.91270557701034E-16,5.64652480907359E-21));
#4497=DIRECTION('center_axis',(5.64652480907605E-21,-2.48267427335009E-18,
1.));
#4498=DIRECTION('ref_axis',(-1.,-9.91270557701034E-16,5.64652480907359E-21));
#4499=DIRECTION('',(-5.64652480907605E-21,2.48267427335009E-18,-1.));
#4500=DIRECTION('center_axis',(5.64652480907605E-21,-2.48267427335009E-18,
1.));
#4501=DIRECTION('ref_axis',(-1.,-9.91270557701034E-16,5.64652480907359E-21));
#4502=DIRECTION('center_axis',(-1.,1.82934475648463E-15,-5.64652480908311E-21));
#4503=DIRECTION('ref_axis',(-1.82934475648463E-15,-1.,2.48267427335006E-18));
#4504=DIRECTION('',(1.82934475648463E-15,1.,-2.48267427335006E-18));
#4505=DIRECTION('',(-5.64652480907605E-21,2.48267427335009E-18,-1.));
#4506=DIRECTION('',(1.82934475648463E-15,1.,-2.48267427335006E-18));
#4507=DIRECTION('center_axis',(-5.64652480907605E-21,2.48267427335009E-18,
-1.));
#4508=DIRECTION('ref_axis',(-1.,-9.91270557701032E-16,5.64652480907359E-21));
#4509=DIRECTION('center_axis',(-5.64652480907605E-21,2.48267427335009E-18,
-1.));
#4510=DIRECTION('ref_axis',(1.,9.91270557701032E-16,-5.64652480907359E-21));
#4511=DIRECTION('',(-5.64652480907605E-21,2.48267427335009E-18,-1.));
#4512=DIRECTION('center_axis',(-5.64652480907605E-21,2.48267427335009E-18,
-1.));
#4513=DIRECTION('ref_axis',(1.,9.91270557701032E-16,-5.64652480907359E-21));
#4514=DIRECTION('center_axis',(1.04083408558608E-15,1.,2.48267427335009E-18));
#4515=DIRECTION('ref_axis',(5.64652480907605E-21,-2.48267427335009E-18,
1.));
#4516=DIRECTION('',(1.,1.04083408558608E-15,5.64652480907598E-21));
#4517=DIRECTION('',(-5.64652480907605E-21,2.48267427335009E-18,-1.));
#4518=DIRECTION('',(1.,1.04083408558608E-15,5.64652480907598E-21));
#4519=DIRECTION('center_axis',(-5.64652480907605E-21,2.48267427335009E-18,
-1.));
#4520=DIRECTION('ref_axis',(-1.,-9.91270557701032E-16,5.64652480907359E-21));
#4521=DIRECTION('center_axis',(5.64652480907605E-21,-2.48267427335009E-18,
1.));
#4522=DIRECTION('ref_axis',(-1.,-9.91270557701032E-16,5.64652480907359E-21));
#4523=DIRECTION('',(-5.64652480907605E-21,2.48267427335009E-18,-1.));
#4524=DIRECTION('center_axis',(5.64652480907605E-21,-2.48267427335009E-18,
1.));
#4525=DIRECTION('ref_axis',(-1.,-9.91270557701032E-16,5.64652480907359E-21));
#4526=DIRECTION('center_axis',(-1.,-1.04083408558608E-15,5.64652480907346E-21));
#4527=DIRECTION('ref_axis',(5.64652480907605E-21,-2.48267427335009E-18,
1.));
#4528=DIRECTION('',(1.04083408558608E-15,1.,-2.48267427335006E-18));
#4529=DIRECTION('',(-5.64652480907605E-21,2.48267427335009E-18,-1.));
#4530=DIRECTION('',(1.04083408558608E-15,1.,-2.48267427335006E-18));
#4531=DIRECTION('center_axis',(-5.64652480907605E-21,2.48267427335009E-18,
-1.));
#4532=DIRECTION('ref_axis',(-1.,-1.98254111540206E-15,5.64652480907113E-21));
#4533=DIRECTION('center_axis',(5.64652480907605E-21,-2.48267427335009E-18,
1.));
#4534=DIRECTION('ref_axis',(-1.,-1.98254111540206E-15,5.64652480907113E-21));
#4535=DIRECTION('',(-5.64652480907605E-21,2.48267427335009E-18,-1.));
#4536=DIRECTION('center_axis',(5.64652480907605E-21,-2.48267427335009E-18,
1.));
#4537=DIRECTION('ref_axis',(-1.,-1.98254111540206E-15,5.64652480907113E-21));
#4538=DIRECTION('center_axis',(6.32663855944483E-16,-1.,2.48267427335006E-18));
#4539=DIRECTION('ref_axis',(1.,6.32663855944483E-16,5.646524809077E-21));
#4540=DIRECTION('',(-1.,-6.32663855944483E-16,-5.646524809077E-21));
#4541=DIRECTION('',(-5.64652480907605E-21,2.48267427335009E-18,-1.));
#4542=DIRECTION('',(-1.,-6.32663855944483E-16,-5.646524809077E-21));
#4543=DIRECTION('center_axis',(-5.64652480907605E-21,2.48267427335009E-18,
-1.));
#4544=DIRECTION('ref_axis',(-1.,-1.98254111540206E-15,5.64652480907113E-21));
#4545=DIRECTION('center_axis',(-5.64652480907605E-21,2.48267427335009E-18,
-1.));
#4546=DIRECTION('ref_axis',(1.,1.98254111540206E-15,-5.64652480907113E-21));
#4547=DIRECTION('',(-5.64652480907605E-21,2.48267427335009E-18,-1.));
#4548=DIRECTION('center_axis',(-5.64652480907605E-21,2.48267427335009E-18,
-1.));
#4549=DIRECTION('ref_axis',(1.,1.98254111540206E-15,-5.64652480907113E-21));
#4550=DIRECTION('center_axis',(-1.,-1.04083408558608E-15,5.64652480907346E-21));
#4551=DIRECTION('ref_axis',(5.64652480907605E-21,-2.48267427335009E-18,
1.));
#4552=DIRECTION('',(1.04083408558608E-15,1.,-2.48267427335006E-18));
#4553=DIRECTION('',(-5.64652480907605E-21,2.48267427335009E-18,-1.));
#4554=DIRECTION('',(1.04083408558608E-15,1.,-2.48267427335006E-18));
#4555=DIRECTION('center_axis',(-5.64652480907605E-21,2.48267427335009E-18,
-1.));
#4556=DIRECTION('ref_axis',(-1.,-1.40184818773261E-38,5.64652480907605E-21));
#4557=DIRECTION('center_axis',(5.64652480907605E-21,-2.48267427335009E-18,
1.));
#4558=DIRECTION('ref_axis',(-1.,-2.80369637546521E-38,5.64652480907605E-21));
#4559=DIRECTION('',(-5.64652480907605E-21,2.48267427335009E-18,-1.));
#4560=DIRECTION('center_axis',(5.64652480907605E-21,-2.48267427335009E-18,
1.));
#4561=DIRECTION('ref_axis',(-1.,-1.40184818773261E-38,5.64652480907605E-21));
#4562=DIRECTION('center_axis',(-1.04083408558608E-15,-1.,-2.48267427335009E-18));
#4563=DIRECTION('ref_axis',(-5.64652480907605E-21,2.48267427335009E-18,
-1.));
#4564=DIRECTION('',(-1.,-1.04083408558608E-15,-5.64652480907598E-21));
#4565=DIRECTION('',(-5.64652480907605E-21,2.48267427335009E-18,-1.));
#4566=DIRECTION('',(-1.,-1.04083408558608E-15,-5.64652480907598E-21));
#4567=DIRECTION('center_axis',(-5.64652480907605E-21,2.48267427335009E-18,
-1.));
#4568=DIRECTION('ref_axis',(-1.,-1.40184818773261E-38,5.64652480907605E-21));
#4569=DIRECTION('center_axis',(5.64652480907605E-21,-2.48267427335009E-18,
1.));
#4570=DIRECTION('ref_axis',(-1.,-2.80369637546521E-38,5.64652480907605E-21));
#4571=DIRECTION('',(-5.64652480907605E-21,2.48267427335009E-18,-1.));
#4572=DIRECTION('center_axis',(5.64652480907605E-21,-2.48267427335009E-18,
1.));
#4573=DIRECTION('ref_axis',(-1.,-1.40184818773261E-38,5.64652480907605E-21));
#4574=DIRECTION('center_axis',(1.,1.04083408558608E-15,-5.64652480907346E-21));
#4575=DIRECTION('ref_axis',(-5.64652480907605E-21,2.48267427335009E-18,
-1.));
#4576=DIRECTION('',(-1.04083408558608E-15,-1.,2.48267427335006E-18));
#4577=DIRECTION('',(-1.04083408558608E-15,-1.,2.48267427335006E-18));
#4578=DIRECTION('center_axis',(5.6465248090734E-21,2.48267427335009E-18,
-1.));
#4579=DIRECTION('ref_axis',(-1.,-1.04083408558608E-15,-5.64652480907598E-21));
#4580=DIRECTION('center_axis',(5.6465248090734E-21,2.48267427335009E-18,
-1.));
#4581=DIRECTION('ref_axis',(-1.,-1.04083408558608E-15,-5.64652480907598E-21));
#5388=CARTESIAN_POINT('',(0.,0.,0.));
#5389=CARTESIAN_POINT('Origin',(11.5,-1.38777878078145E-14,1.5));
#5390=CARTESIAN_POINT('',(11.5,-1.38802704820878E-14,0.50000000000001));
#5391=CARTESIAN_POINT('Origin',(11.5,-1.38777878078145E-14,1.5));
#5392=CARTESIAN_POINT('',(11.5,23.1,0.50000000000001));
#5393=CARTESIAN_POINT('',(11.5,-1.38802704820878E-14,0.50000000000001));
#5394=CARTESIAN_POINT('Origin',(11.5,23.1,1.5));
#5395=CARTESIAN_POINT('Origin',(11.5,-1.38777878078145E-14,1.5));
#5396=CARTESIAN_POINT('',(11.5,53.1,0.50000000000001));
#5397=CARTESIAN_POINT('Origin',(11.5,53.1,1.5));
#5398=CARTESIAN_POINT('',(11.5000000000001,76.2,0.50000000000001));
#5399=CARTESIAN_POINT('',(11.5,-1.38802704820878E-14,0.50000000000001));
#5400=CARTESIAN_POINT('Origin',(11.5,76.2,1.5));
#5401=CARTESIAN_POINT('Origin',(50.5,7.63278329429795E-14,1.5));
#5402=CARTESIAN_POINT('',(51.5,24.6000000000001,1.5));
#5403=CARTESIAN_POINT('Origin',(50.5,24.6000000000001,1.5));
#5404=CARTESIAN_POINT('',(51.5000000000001,51.6000000000001,1.5));
#5405=CARTESIAN_POINT('',(51.5,7.48788286277518E-14,1.5));
#5406=CARTESIAN_POINT('Origin',(50.5000000000001,51.6000000000001,1.5));
#5407=CARTESIAN_POINT('Origin',(3.5,56.6,2.99999999999995));
#5408=CARTESIAN_POINT('',(0.,56.6,0.));
#5409=CARTESIAN_POINT('',(3.50000000000003,53.1,0.));
#5410=CARTESIAN_POINT('Origin',(3.5,56.6,0.));
#5411=CARTESIAN_POINT('',(3.50000000000003,53.1,2.99999999999995));
#5412=CARTESIAN_POINT('',(3.50000000000003,53.1,2.99999999999995));
#5413=CARTESIAN_POINT('',(0.,56.6,2.99999999999995));
#5414=CARTESIAN_POINT('Origin',(3.5,56.6,2.99999999999995));
#5415=CARTESIAN_POINT('',(0.,56.6,2.99999999999995));
#5416=CARTESIAN_POINT('Origin',(21.5,53.1000000000001,2.99999999999995));
#5417=CARTESIAN_POINT('',(21.5,53.1000000000001,0.));
#5418=CARTESIAN_POINT('',(21.5,53.1000000000001,0.));
#5419=CARTESIAN_POINT('',(21.5,53.1000000000001,2.99999999999995));
#5420=CARTESIAN_POINT('',(21.5,53.1000000000001,2.99999999999995));
#5421=CARTESIAN_POINT('',(21.5,53.1000000000001,2.99999999999995));
#5422=CARTESIAN_POINT('Origin',(21.5,49.6000000000001,2.99999999999995));
#5423=CARTESIAN_POINT('',(25.,49.6,0.));
#5424=CARTESIAN_POINT('Origin',(21.5,49.6000000000001,0.));
#5425=CARTESIAN_POINT('',(25.,49.6,2.99999999999995));
#5426=CARTESIAN_POINT('',(25.,49.6,2.99999999999995));
#5427=CARTESIAN_POINT('Origin',(21.5,49.6000000000001,2.99999999999995));
#5428=CARTESIAN_POINT('Origin',(25.0000000000001,26.6000000000001,2.99999999999995));
#5429=CARTESIAN_POINT('',(25.0000000000001,26.6000000000001,0.));
#5430=CARTESIAN_POINT('',(25.0000000000001,26.6000000000001,0.));
#5431=CARTESIAN_POINT('',(25.0000000000001,26.6000000000001,2.99999999999995));
#5432=CARTESIAN_POINT('',(25.0000000000001,26.6000000000001,2.99999999999995));
#5433=CARTESIAN_POINT('',(25.0000000000001,26.6000000000001,2.99999999999995));
#5434=CARTESIAN_POINT('Origin',(21.5000000000001,26.6,2.99999999999995));
#5435=CARTESIAN_POINT('',(21.5,23.1,0.));
#5436=CARTESIAN_POINT('Origin',(21.5000000000001,26.6,0.));
#5437=CARTESIAN_POINT('',(21.5,23.1,2.99999999999995));
#5438=CARTESIAN_POINT('',(21.5,23.1,2.99999999999995));
#5439=CARTESIAN_POINT('Origin',(21.5000000000001,26.6,2.99999999999995));
#5440=CARTESIAN_POINT('Origin',(3.50000000000009,23.1,2.99999999999995));
#5441=CARTESIAN_POINT('',(3.50000000000009,23.1,0.));
#5442=CARTESIAN_POINT('',(3.50000000000009,23.1,0.));
#5443=CARTESIAN_POINT('',(3.50000000000009,23.1,2.99999999999995));
#5444=CARTESIAN_POINT('',(3.50000000000009,23.1,2.99999999999995));
#5445=CARTESIAN_POINT('',(3.50000000000009,23.1,2.99999999999995));
#5446=CARTESIAN_POINT('Origin',(3.50000000000006,19.6,2.99999999999995));
#5447=CARTESIAN_POINT('',(4.16333634234434E-14,19.6,0.));
#5448=CARTESIAN_POINT('Origin',(3.50000000000006,19.6,0.));
#5449=CARTESIAN_POINT('',(4.16333634234434E-14,19.6,2.99999999999995));
#5450=CARTESIAN_POINT('',(4.16333634234434E-14,19.6,2.99999999999995));
#5451=CARTESIAN_POINT('Origin',(3.50000000000006,19.6,2.99999999999995));
#5452=CARTESIAN_POINT('Origin',(0.,3.50000000000002,2.99999999999995));
#5453=CARTESIAN_POINT('',(0.,3.50000000000002,0.));
#5454=CARTESIAN_POINT('',(0.,3.50000000000002,0.));
#5455=CARTESIAN_POINT('',(0.,3.50000000000002,2.99999999999995));
#5456=CARTESIAN_POINT('',(0.,3.50000000000002,2.99999999999995));
#5457=CARTESIAN_POINT('',(0.,3.50000000000002,2.99999999999995));
#5458=CARTESIAN_POINT('Origin',(3.49999999999999,3.5,2.99999999999995));
#5459=CARTESIAN_POINT('',(3.50000000000002,0.,0.));
#5460=CARTESIAN_POINT('Origin',(3.49999999999999,3.5,0.));
#5461=CARTESIAN_POINT('',(3.50000000000002,0.,2.99999999999995));
#5462=CARTESIAN_POINT('',(3.50000000000002,0.,2.99999999999995));
#5463=CARTESIAN_POINT('Origin',(3.49999999999999,3.5,2.99999999999995));
#5464=CARTESIAN_POINT('Origin',(34.5,2.77555756156289E-14,2.99999999999995));
#5465=CARTESIAN_POINT('',(34.5,2.77555756156289E-14,0.));
#5466=CARTESIAN_POINT('',(34.5,2.77555756156289E-14,0.));
#5467=CARTESIAN_POINT('',(34.5,2.77555756156289E-14,2.99999999999995));
#5468=CARTESIAN_POINT('',(34.5,2.77555756156289E-14,2.99999999999995));
#5469=CARTESIAN_POINT('',(34.5,2.77555756156289E-14,2.99999999999995));
#5470=CARTESIAN_POINT('Origin',(34.5,3.50000000000003,2.99999999999995));
#5471=CARTESIAN_POINT('',(38.,3.5,0.));
#5472=CARTESIAN_POINT('Origin',(34.5,3.50000000000003,0.));
#5473=CARTESIAN_POINT('',(38.,3.5,2.99999999999995));
#5474=CARTESIAN_POINT('',(38.,3.5,2.99999999999995));
#5475=CARTESIAN_POINT('Origin',(34.5,3.50000000000003,2.99999999999995));
#5476=CARTESIAN_POINT('Origin',(38.0000000000001,21.1,2.99999999999995));
#5477=CARTESIAN_POINT('',(38.0000000000001,21.1,0.));
#5478=CARTESIAN_POINT('',(38.0000000000001,21.1,0.));
#5479=CARTESIAN_POINT('',(38.0000000000001,21.1,2.99999999999995));
#5480=CARTESIAN_POINT('',(38.0000000000001,21.1,2.99999999999995));
#5481=CARTESIAN_POINT('',(38.0000000000001,21.1,2.99999999999995));
#5482=CARTESIAN_POINT('Origin',(41.5000000000001,21.1000000000001,2.99999999999995));
#5483=CARTESIAN_POINT('',(41.5,24.6000000000001,0.));
#5484=CARTESIAN_POINT('Origin',(41.5000000000001,21.1000000000001,0.));
#5485=CARTESIAN_POINT('',(41.5,24.6000000000001,2.99999999999995));
#5486=CARTESIAN_POINT('',(41.5,24.6000000000001,2.99999999999995));
#5487=CARTESIAN_POINT('Origin',(41.5000000000001,21.1000000000001,2.99999999999995));
#5488=CARTESIAN_POINT('Origin',(58.5,24.6000000000001,2.99999999999995));
#5489=CARTESIAN_POINT('',(58.5,24.6000000000001,0.));
#5490=CARTESIAN_POINT('',(58.5,24.6000000000001,0.));
#5491=CARTESIAN_POINT('',(58.5,24.6000000000001,2.99999999999995));
#5492=CARTESIAN_POINT('',(58.5,24.6000000000001,2.99999999999995));
#5493=CARTESIAN_POINT('',(58.5,24.6000000000001,2.99999999999995));
#5494=CARTESIAN_POINT('Origin',(58.5,28.1000000000001,2.99999999999995));
#5495=CARTESIAN_POINT('',(62.,28.1000000000001,0.));
#5496=CARTESIAN_POINT('Origin',(58.5,28.1000000000001,0.));
#5497=CARTESIAN_POINT('',(62.,28.1000000000001,2.99999999999995));
#5498=CARTESIAN_POINT('',(62.,28.1000000000001,2.99999999999995));
#5499=CARTESIAN_POINT('Origin',(58.5,28.1000000000001,2.99999999999995));
#5500=CARTESIAN_POINT('Origin',(62.,48.1000000000001,2.99999999999995));
#5501=CARTESIAN_POINT('',(62.,48.1000000000001,0.));
#5502=CARTESIAN_POINT('',(62.,48.1000000000001,0.));
#5503=CARTESIAN_POINT('',(62.,48.1000000000001,2.99999999999995));
#5504=CARTESIAN_POINT('',(62.,48.1000000000001,2.99999999999995));
#5505=CARTESIAN_POINT('',(62.,48.1000000000001,2.99999999999995));
#5506=CARTESIAN_POINT('Origin',(58.5,48.1000000000001,2.99999999999995));
#5507=CARTESIAN_POINT('',(58.5,51.6000000000001,0.));
#5508=CARTESIAN_POINT('Origin',(58.5,48.1000000000001,0.));
#5509=CARTESIAN_POINT('',(58.5,51.6000000000001,2.99999999999995));
#5510=CARTESIAN_POINT('',(58.5,51.6000000000001,2.99999999999995));
#5511=CARTESIAN_POINT('Origin',(58.5,48.1000000000001,2.99999999999995));
#5512=CARTESIAN_POINT('Origin',(41.5,51.6,2.99999999999995));
#5513=CARTESIAN_POINT('',(41.5,51.6,0.));
#5514=CARTESIAN_POINT('',(41.5,51.6,0.));
#5515=CARTESIAN_POINT('',(41.5,51.6,2.99999999999995));
#5516=CARTESIAN_POINT('',(41.5,51.6,2.99999999999995));
#5517=CARTESIAN_POINT('',(41.5,51.6,2.99999999999995));
#5518=CARTESIAN_POINT('Origin',(41.5,55.1,2.99999999999995));
#5519=CARTESIAN_POINT('',(38.,55.1,0.));
#5520=CARTESIAN_POINT('Origin',(41.5,55.1,0.));
#5521=CARTESIAN_POINT('',(38.,55.1,2.99999999999995));
#5522=CARTESIAN_POINT('',(38.,55.1,2.99999999999995));
#5523=CARTESIAN_POINT('Origin',(41.5,55.1,2.99999999999995));
#5524=CARTESIAN_POINT('Origin',(38.,72.7,2.99999999999995));
#5525=CARTESIAN_POINT('',(38.,72.7,0.));
#5526=CARTESIAN_POINT('',(38.,72.7,0.));
#5527=CARTESIAN_POINT('',(38.,72.7,2.99999999999995));
#5528=CARTESIAN_POINT('',(38.,72.7,2.99999999999995));
#5529=CARTESIAN_POINT('',(38.,72.7,2.99999999999995));
#5530=CARTESIAN_POINT('Origin',(34.5,72.7000000000001,2.99999999999995));
#5531=CARTESIAN_POINT('',(34.5,76.2000000000001,0.));
#5532=CARTESIAN_POINT('Origin',(34.5,72.7000000000001,0.));
#5533=CARTESIAN_POINT('',(34.5,76.2000000000001,2.99999999999995));
#5534=CARTESIAN_POINT('',(34.5,76.2000000000001,2.99999999999995));
#5535=CARTESIAN_POINT('Origin',(34.5,72.7000000000001,2.99999999999995));
#5536=CARTESIAN_POINT('Origin',(3.50000000000009,76.2,2.99999999999995));
#5537=CARTESIAN_POINT('',(3.50000000000009,76.2,0.));
#5538=CARTESIAN_POINT('',(3.50000000000009,76.2,0.));
#5539=CARTESIAN_POINT('',(3.50000000000009,76.2,2.99999999999995));
#5540=CARTESIAN_POINT('',(3.50000000000009,76.2,2.99999999999995));
#5541=CARTESIAN_POINT('',(3.50000000000009,76.2,2.99999999999995));
#5542=CARTESIAN_POINT('Origin',(3.5000000000001,72.7,2.99999999999995));
#5543=CARTESIAN_POINT('',(4.16333634234434E-14,72.7,0.));
#5544=CARTESIAN_POINT('Origin',(3.5000000000001,72.7,0.));
#5545=CARTESIAN_POINT('',(4.16333634234434E-14,72.7,2.99999999999995));
#5546=CARTESIAN_POINT('',(4.16333634234434E-14,72.7,2.99999999999995));
#5547=CARTESIAN_POINT('Origin',(3.5000000000001,72.7,2.99999999999995));
#5548=CARTESIAN_POINT('Origin',(0.,56.6,2.99999999999995));
#5549=CARTESIAN_POINT('',(0.,56.6,0.));
#5550=CARTESIAN_POINT('',(0.,56.6,2.99999999999995));
#5551=CARTESIAN_POINT('Origin',(3.5,56.6,2.99999999999995));
#5552=CARTESIAN_POINT('Origin',(3.5,56.6,0.));
#5589=UNCERTAINTY_MEASURE_WITH_UNIT(LENGTH_MEASURE(0.01),#5600,
'DISTANCE_ACCURACY_VALUE',
'Maximum model space distance between geometric entities at asserted c
onnectivities');
#5591=UNCERTAINTY_MEASURE_WITH_UNIT(LENGTH_MEASURE(0.01),#5600,
'DISTANCE_ACCURACY_VALUE',
'Maximum model space distance between geometric entities at asserted c
onnectivities');
#5597=(
GEOMETRIC_REPRESENTATION_CONTEXT(3)
GLOBAL_UNCERTAINTY_ASSIGNED_CONTEXT((#5589))
GLOBAL_UNIT_ASSIGNED_CONTEXT((#5600,#5602,#5603))
REPRESENTATION_CONTEXT('','3D')
);
#5599=(
GEOMETRIC_REPRESENTATION_CONTEXT(3)
GLOBAL_UNCERTAINTY_ASSIGNED_CONTEXT((#5591))
GLOBAL_UNIT_ASSIGNED_CONTEXT((#5600,#5602,#5603))
REPRESENTATION_CONTEXT('','3D')
);
#5600=(
LENGTH_UNIT()
NAMED_UNIT(*)
SI_UNIT(.MILLI.,.METRE.)
);
#5602=(
NAMED_UNIT(*)
PLANE_ANGLE_UNIT()
SI_UNIT($,.RADIAN.)
);
#5603=(
NAMED_UNIT(*)
SI_UNIT($,.STERADIAN.)
SOLID_ANGLE_UNIT()
);
#5609=SHAPE_DEFINITION_REPRESENTATION(#5616,#5645);
#5616=PRODUCT_DEFINITION_SHAPE('',$,#5653);
#5645=SHAPE_REPRESENTATION('',(#3593),#5597);
#5647=PRODUCT_DEFINITION_CONTEXT('part definition',#5670,'design');
#5653=PRODUCT_DEFINITION('Link','Link',#5660,#5647);
#5660=PRODUCT_DEFINITION_FORMATION('',$,#5677);
#5670=APPLICATION_CONTEXT(
'Core Data for Automotive Mechanical Design Process');
#5671=PRODUCT_CONTEXT('part definition',#5670,'mechanical');
#5677=PRODUCT('Link','Link',$,(#5671));
#5680=PRESENTATION_STYLE_ASSIGNMENT((#5683));
#5683=SURFACE_STYLE_USAGE(.BOTH.,#5686);
#5686=SURFACE_SIDE_STYLE('',(#5689));
#5689=SURFACE_STYLE_FILL_AREA(#5692);
#5692=FILL_AREA_STYLE('Opaque(97,158,199)',(#5695));
#5695=FILL_AREA_STYLE_COLOUR('Opaque(97,158,199)',#5698);
#5698=COLOUR_RGB('Opaque(97,158,199)',0.380392156862745,0.619607843137255,
0.780392156862745);
ENDSEC;
END-ISO-10303-21;
